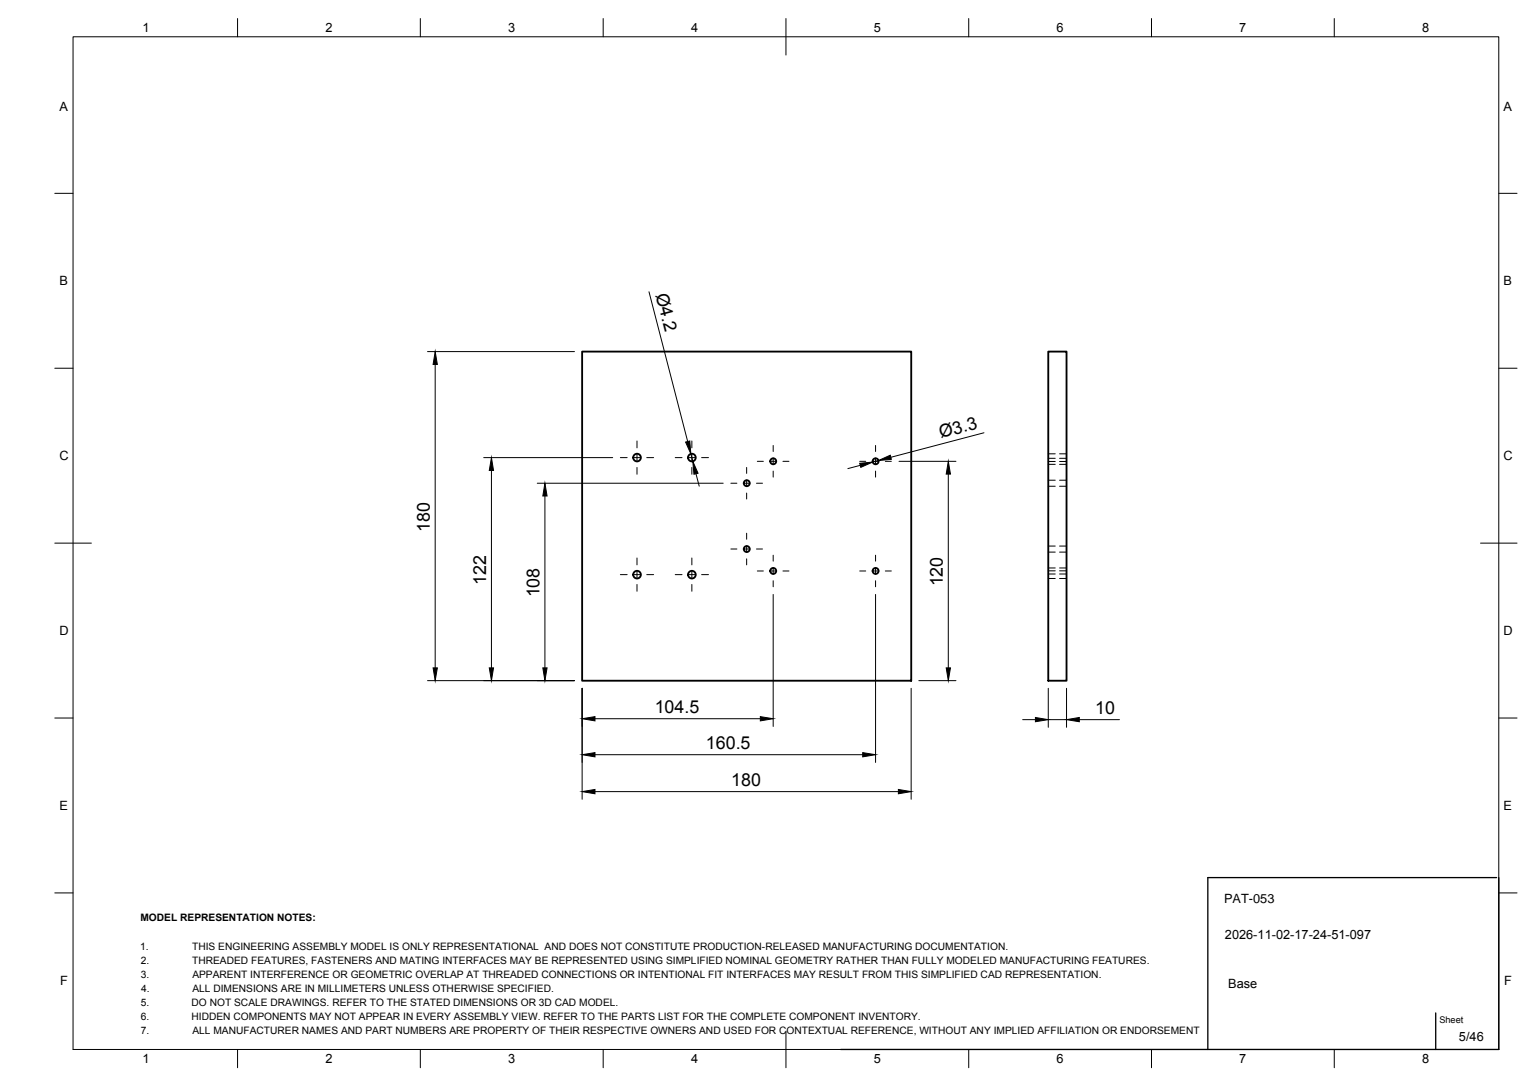
ISO-10303-21;
HEADER;
/* Generated by software containing ST-Developer
 * from STEP Tools, Inc. (www.steptools.com) 
 */

FILE_DESCRIPTION(
/* description */ ('Hand-operated arbor press'),
/* implementation_level */ '2;1');

FILE_NAME(
/* name */ 'Base.step',
/* time_stamp */ '2026-10-28T03:25:25-07:00',
/* author */ (''),
/* organization */ (''),
/* preprocessor_version */ 'ST-DEVELOPER v20.2',
/* originating_system */ 'Autodesk Translation Framework v15.17.0.0',
/* authorisation */ '');

FILE_SCHEMA (('AUTOMOTIVE_DESIGN { 1 0 10303 214 3 1 1 }'));
ENDSEC;

DATA;
#10=MECHANICAL_DESIGN_GEOMETRIC_PRESENTATION_REPRESENTATION('',(#586),#32751);
#502=SHAPE_REPRESENTATION_RELATIONSHIP('SRR','None',#32931,#544);
#544=ADVANCED_BREP_SHAPE_REPRESENTATION('',(#635),#32705);
#586=STYLED_ITEM('',(#33221),#635);
#635=MANIFOLD_SOLID_BREP('Body1',#12483);
#680=FACE_BOUND('',#1989,.T.);
#681=FACE_BOUND('',#1990,.T.);
#682=FACE_BOUND('',#1991,.T.);
#683=FACE_BOUND('',#1992,.T.);
#684=FACE_BOUND('',#1993,.T.);
#685=FACE_BOUND('',#1994,.T.);
#686=FACE_BOUND('',#1995,.T.);
#687=FACE_BOUND('',#1996,.T.);
#688=FACE_BOUND('',#1997,.T.);
#689=FACE_BOUND('',#1998,.T.);
#690=FACE_BOUND('',#2000,.T.);
#691=FACE_BOUND('',#2001,.T.);
#692=FACE_BOUND('',#2002,.T.);
#693=FACE_BOUND('',#2003,.T.);
#694=FACE_BOUND('',#2004,.T.);
#695=FACE_BOUND('',#2005,.T.);
#696=FACE_BOUND('',#2006,.T.);
#697=FACE_BOUND('',#2007,.T.);
#698=FACE_BOUND('',#2008,.T.);
#699=FACE_BOUND('',#2009,.T.);
#849=PLANE('',#13032);
#850=PLANE('',#13033);
#851=PLANE('',#13034);
#852=PLANE('',#13035);
#853=PLANE('',#13036);
#854=PLANE('',#13037);
#1293=FACE_OUTER_BOUND('',#1974,.T.);
#1294=FACE_OUTER_BOUND('',#1975,.T.);
#1295=FACE_OUTER_BOUND('',#1976,.T.);
#1296=FACE_OUTER_BOUND('',#1977,.T.);
#1297=FACE_OUTER_BOUND('',#1978,.T.);
#1298=FACE_OUTER_BOUND('',#1979,.T.);
#1299=FACE_OUTER_BOUND('',#1980,.T.);
#1300=FACE_OUTER_BOUND('',#1981,.T.);
#1301=FACE_OUTER_BOUND('',#1982,.T.);
#1302=FACE_OUTER_BOUND('',#1983,.T.);
#1303=FACE_OUTER_BOUND('',#1984,.T.);
#1304=FACE_OUTER_BOUND('',#1985,.T.);
#1305=FACE_OUTER_BOUND('',#1986,.T.);
#1306=FACE_OUTER_BOUND('',#1987,.T.);
#1307=FACE_OUTER_BOUND('',#1988,.T.);
#1308=FACE_OUTER_BOUND('',#1999,.T.);
#1974=EDGE_LOOP('',(#8324,#8325,#8326,#8327));
#1975=EDGE_LOOP('',(#8328,#8329,#8330,#8331));
#1976=EDGE_LOOP('',(#8332,#8333,#8334,#8335));
#1977=EDGE_LOOP('',(#8336,#8337,#8338,#8339));
#1978=EDGE_LOOP('',(#8340,#8341,#8342,#8343));
#1979=EDGE_LOOP('',(#8344,#8345,#8346,#8347));
#1980=EDGE_LOOP('',(#8348,#8349,#8350,#8351));
#1981=EDGE_LOOP('',(#8352,#8353,#8354,#8355));
#1982=EDGE_LOOP('',(#8356,#8357,#8358,#8359));
#1983=EDGE_LOOP('',(#8360,#8361,#8362,#8363));
#1984=EDGE_LOOP('',(#8364,#8365,#8366,#8367));
#1985=EDGE_LOOP('',(#8368,#8369,#8370,#8371));
#1986=EDGE_LOOP('',(#8372,#8373,#8374,#8375));
#1987=EDGE_LOOP('',(#8376,#8377,#8378,#8379));
#1988=EDGE_LOOP('',(#8380,#8381,#8382,#8383));
#1989=EDGE_LOOP('',(#8384));
#1990=EDGE_LOOP('',(#8385));
#1991=EDGE_LOOP('',(#8386));
#1992=EDGE_LOOP('',(#8387));
#1993=EDGE_LOOP('',(#8388));
#1994=EDGE_LOOP('',(#8389));
#1995=EDGE_LOOP('',(#8390));
#1996=EDGE_LOOP('',(#8391));
#1997=EDGE_LOOP('',(#8392));
#1998=EDGE_LOOP('',(#8393));
#1999=EDGE_LOOP('',(#8394,#8395,#8396,#8397));
#2000=EDGE_LOOP('',(#8398));
#2001=EDGE_LOOP('',(#8399));
#2002=EDGE_LOOP('',(#8400));
#2003=EDGE_LOOP('',(#8401));
#2004=EDGE_LOOP('',(#8402));
#2005=EDGE_LOOP('',(#8403));
#2006=EDGE_LOOP('',(#8404));
#2007=EDGE_LOOP('',(#8405));
#2008=EDGE_LOOP('',(#8406));
#2009=EDGE_LOOP('',(#8407));
#2824=LINE('',#17645,#3995);
#2825=LINE('',#17651,#3996);
#2826=LINE('',#17657,#3997);
#2827=LINE('',#17663,#3998);
#2828=LINE('',#17669,#3999);
#2829=LINE('',#17675,#4000);
#2830=LINE('',#17681,#4001);
#2831=LINE('',#17687,#4002);
#2832=LINE('',#17693,#4003);
#2833=LINE('',#17699,#4004);
#2834=LINE('',#17704,#4005);
#2835=LINE('',#17706,#4006);
#2836=LINE('',#17708,#4007);
#2837=LINE('',#17709,#4008);
#2838=LINE('',#17712,#4009);
#2839=LINE('',#17714,#4010);
#2840=LINE('',#17715,#4011);
#2841=LINE('',#17718,#4012);
#2842=LINE('',#17720,#4013);
#2843=LINE('',#17721,#4014);
#2844=LINE('',#17723,#4015);
#2845=LINE('',#17724,#4016);
#3995=VECTOR('',#14165,0.165);
#3996=VECTOR('',#14172,0.165);
#3997=VECTOR('',#14179,0.165);
#3998=VECTOR('',#14186,0.165);
#3999=VECTOR('',#14193,0.165);
#4000=VECTOR('',#14200,0.165);
#4001=VECTOR('',#14207,0.21);
#4002=VECTOR('',#14214,0.21);
#4003=VECTOR('',#14221,0.21);
#4004=VECTOR('',#14228,0.21);
#4005=VECTOR('',#14233,1.);
#4006=VECTOR('',#14234,1.);
#4007=VECTOR('',#14235,1.);
#4008=VECTOR('',#14236,1.);
#4009=VECTOR('',#14239,1.);
#4010=VECTOR('',#14240,1.);
#4011=VECTOR('',#14241,1.);
#4012=VECTOR('',#14244,1.);
#4013=VECTOR('',#14245,1.);
#4014=VECTOR('',#14246,1.);
#4015=VECTOR('',#14249,1.);
#4016=VECTOR('',#14250,1.);
#5166=CIRCLE('',#13003,0.165);
#5167=CIRCLE('',#13004,0.165);
#5168=CIRCLE('',#13006,0.165);
#5169=CIRCLE('',#13007,0.165);
#5170=CIRCLE('',#13009,0.165);
#5171=CIRCLE('',#13010,0.165);
#5172=CIRCLE('',#13012,0.165);
#5173=CIRCLE('',#13013,0.165);
#5174=CIRCLE('',#13015,0.165);
#5175=CIRCLE('',#13016,0.165);
#5176=CIRCLE('',#13018,0.165);
#5177=CIRCLE('',#13019,0.165);
#5178=CIRCLE('',#13021,0.21);
#5179=CIRCLE('',#13022,0.21);
#5180=CIRCLE('',#13024,0.21);
#5181=CIRCLE('',#13025,0.21);
#5182=CIRCLE('',#13027,0.21);
#5183=CIRCLE('',#13028,0.21);
#5184=CIRCLE('',#13030,0.21);
#5185=CIRCLE('',#13031,0.21);
#5556=VERTEX_POINT('',#17642);
#5557=VERTEX_POINT('',#17644);
#5558=VERTEX_POINT('',#17648);
#5559=VERTEX_POINT('',#17650);
#5560=VERTEX_POINT('',#17654);
#5561=VERTEX_POINT('',#17656);
#5562=VERTEX_POINT('',#17660);
#5563=VERTEX_POINT('',#17662);
#5564=VERTEX_POINT('',#17666);
#5565=VERTEX_POINT('',#17668);
#5566=VERTEX_POINT('',#17672);
#5567=VERTEX_POINT('',#17674);
#5568=VERTEX_POINT('',#17678);
#5569=VERTEX_POINT('',#17680);
#5570=VERTEX_POINT('',#17684);
#5571=VERTEX_POINT('',#17686);
#5572=VERTEX_POINT('',#17690);
#5573=VERTEX_POINT('',#17692);
#5574=VERTEX_POINT('',#17696);
#5575=VERTEX_POINT('',#17698);
#5576=VERTEX_POINT('',#17702);
#5577=VERTEX_POINT('',#17703);
#5578=VERTEX_POINT('',#17705);
#5579=VERTEX_POINT('',#17707);
#5580=VERTEX_POINT('',#17711);
#5581=VERTEX_POINT('',#17713);
#5582=VERTEX_POINT('',#17717);
#5583=VERTEX_POINT('',#17719);
#6665=EDGE_CURVE('',#5556,#5556,#5166,.T.);
#6666=EDGE_CURVE('',#5556,#5557,#2824,.T.);
#6667=EDGE_CURVE('',#5557,#5557,#5167,.T.);
#6668=EDGE_CURVE('',#5558,#5558,#5168,.T.);
#6669=EDGE_CURVE('',#5558,#5559,#2825,.T.);
#6670=EDGE_CURVE('',#5559,#5559,#5169,.T.);
#6671=EDGE_CURVE('',#5560,#5560,#5170,.T.);
#6672=EDGE_CURVE('',#5560,#5561,#2826,.T.);
#6673=EDGE_CURVE('',#5561,#5561,#5171,.T.);
#6674=EDGE_CURVE('',#5562,#5562,#5172,.T.);
#6675=EDGE_CURVE('',#5562,#5563,#2827,.T.);
#6676=EDGE_CURVE('',#5563,#5563,#5173,.T.);
#6677=EDGE_CURVE('',#5564,#5564,#5174,.T.);
#6678=EDGE_CURVE('',#5564,#5565,#2828,.T.);
#6679=EDGE_CURVE('',#5565,#5565,#5175,.T.);
#6680=EDGE_CURVE('',#5566,#5566,#5176,.T.);
#6681=EDGE_CURVE('',#5566,#5567,#2829,.T.);
#6682=EDGE_CURVE('',#5567,#5567,#5177,.T.);
#6683=EDGE_CURVE('',#5568,#5568,#5178,.T.);
#6684=EDGE_CURVE('',#5568,#5569,#2830,.T.);
#6685=EDGE_CURVE('',#5569,#5569,#5179,.T.);
#6686=EDGE_CURVE('',#5570,#5570,#5180,.T.);
#6687=EDGE_CURVE('',#5570,#5571,#2831,.T.);
#6688=EDGE_CURVE('',#5571,#5571,#5181,.T.);
#6689=EDGE_CURVE('',#5572,#5572,#5182,.T.);
#6690=EDGE_CURVE('',#5572,#5573,#2832,.T.);
#6691=EDGE_CURVE('',#5573,#5573,#5183,.T.);
#6692=EDGE_CURVE('',#5574,#5574,#5184,.T.);
#6693=EDGE_CURVE('',#5574,#5575,#2833,.T.);
#6694=EDGE_CURVE('',#5575,#5575,#5185,.T.);
#6695=EDGE_CURVE('',#5576,#5577,#2834,.T.);
#6696=EDGE_CURVE('',#5577,#5578,#2835,.T.);
#6697=EDGE_CURVE('',#5579,#5578,#2836,.T.);
#6698=EDGE_CURVE('',#5576,#5579,#2837,.T.);
#6699=EDGE_CURVE('',#5580,#5576,#2838,.T.);
#6700=EDGE_CURVE('',#5581,#5579,#2839,.T.);
#6701=EDGE_CURVE('',#5580,#5581,#2840,.T.);
#6702=EDGE_CURVE('',#5582,#5580,#2841,.T.);
#6703=EDGE_CURVE('',#5583,#5581,#2842,.T.);
#6704=EDGE_CURVE('',#5582,#5583,#2843,.T.);
#6705=EDGE_CURVE('',#5577,#5582,#2844,.T.);
#6706=EDGE_CURVE('',#5578,#5583,#2845,.T.);
#8324=ORIENTED_EDGE('',*,*,#6665,.F.);
#8325=ORIENTED_EDGE('',*,*,#6666,.T.);
#8326=ORIENTED_EDGE('',*,*,#6667,.F.);
#8327=ORIENTED_EDGE('',*,*,#6666,.F.);
#8328=ORIENTED_EDGE('',*,*,#6668,.F.);
#8329=ORIENTED_EDGE('',*,*,#6669,.T.);
#8330=ORIENTED_EDGE('',*,*,#6670,.F.);
#8331=ORIENTED_EDGE('',*,*,#6669,.F.);
#8332=ORIENTED_EDGE('',*,*,#6671,.F.);
#8333=ORIENTED_EDGE('',*,*,#6672,.T.);
#8334=ORIENTED_EDGE('',*,*,#6673,.F.);
#8335=ORIENTED_EDGE('',*,*,#6672,.F.);
#8336=ORIENTED_EDGE('',*,*,#6674,.F.);
#8337=ORIENTED_EDGE('',*,*,#6675,.T.);
#8338=ORIENTED_EDGE('',*,*,#6676,.F.);
#8339=ORIENTED_EDGE('',*,*,#6675,.F.);
#8340=ORIENTED_EDGE('',*,*,#6677,.F.);
#8341=ORIENTED_EDGE('',*,*,#6678,.T.);
#8342=ORIENTED_EDGE('',*,*,#6679,.F.);
#8343=ORIENTED_EDGE('',*,*,#6678,.F.);
#8344=ORIENTED_EDGE('',*,*,#6680,.F.);
#8345=ORIENTED_EDGE('',*,*,#6681,.T.);
#8346=ORIENTED_EDGE('',*,*,#6682,.F.);
#8347=ORIENTED_EDGE('',*,*,#6681,.F.);
#8348=ORIENTED_EDGE('',*,*,#6683,.F.);
#8349=ORIENTED_EDGE('',*,*,#6684,.T.);
#8350=ORIENTED_EDGE('',*,*,#6685,.F.);
#8351=ORIENTED_EDGE('',*,*,#6684,.F.);
#8352=ORIENTED_EDGE('',*,*,#6686,.F.);
#8353=ORIENTED_EDGE('',*,*,#6687,.T.);
#8354=ORIENTED_EDGE('',*,*,#6688,.F.);
#8355=ORIENTED_EDGE('',*,*,#6687,.F.);
#8356=ORIENTED_EDGE('',*,*,#6689,.F.);
#8357=ORIENTED_EDGE('',*,*,#6690,.T.);
#8358=ORIENTED_EDGE('',*,*,#6691,.F.);
#8359=ORIENTED_EDGE('',*,*,#6690,.F.);
#8360=ORIENTED_EDGE('',*,*,#6692,.F.);
#8361=ORIENTED_EDGE('',*,*,#6693,.T.);
#8362=ORIENTED_EDGE('',*,*,#6694,.F.);
#8363=ORIENTED_EDGE('',*,*,#6693,.F.);
#8364=ORIENTED_EDGE('',*,*,#6695,.T.);
#8365=ORIENTED_EDGE('',*,*,#6696,.T.);
#8366=ORIENTED_EDGE('',*,*,#6697,.F.);
#8367=ORIENTED_EDGE('',*,*,#6698,.F.);
#8368=ORIENTED_EDGE('',*,*,#6699,.T.);
#8369=ORIENTED_EDGE('',*,*,#6698,.T.);
#8370=ORIENTED_EDGE('',*,*,#6700,.F.);
#8371=ORIENTED_EDGE('',*,*,#6701,.F.);
#8372=ORIENTED_EDGE('',*,*,#6702,.T.);
#8373=ORIENTED_EDGE('',*,*,#6701,.T.);
#8374=ORIENTED_EDGE('',*,*,#6703,.F.);
#8375=ORIENTED_EDGE('',*,*,#6704,.F.);
#8376=ORIENTED_EDGE('',*,*,#6705,.T.);
#8377=ORIENTED_EDGE('',*,*,#6704,.T.);
#8378=ORIENTED_EDGE('',*,*,#6706,.F.);
#8379=ORIENTED_EDGE('',*,*,#6696,.F.);
#8380=ORIENTED_EDGE('',*,*,#6706,.T.);
#8381=ORIENTED_EDGE('',*,*,#6703,.T.);
#8382=ORIENTED_EDGE('',*,*,#6700,.T.);
#8383=ORIENTED_EDGE('',*,*,#6697,.T.);
#8384=ORIENTED_EDGE('',*,*,#6673,.T.);
#8385=ORIENTED_EDGE('',*,*,#6676,.T.);
#8386=ORIENTED_EDGE('',*,*,#6679,.T.);
#8387=ORIENTED_EDGE('',*,*,#6682,.T.);
#8388=ORIENTED_EDGE('',*,*,#6685,.T.);
#8389=ORIENTED_EDGE('',*,*,#6688,.T.);
#8390=ORIENTED_EDGE('',*,*,#6691,.T.);
#8391=ORIENTED_EDGE('',*,*,#6694,.T.);
#8392=ORIENTED_EDGE('',*,*,#6670,.T.);
#8393=ORIENTED_EDGE('',*,*,#6667,.T.);
#8394=ORIENTED_EDGE('',*,*,#6705,.F.);
#8395=ORIENTED_EDGE('',*,*,#6695,.F.);
#8396=ORIENTED_EDGE('',*,*,#6699,.F.);
#8397=ORIENTED_EDGE('',*,*,#6702,.F.);
#8398=ORIENTED_EDGE('',*,*,#6671,.T.);
#8399=ORIENTED_EDGE('',*,*,#6674,.T.);
#8400=ORIENTED_EDGE('',*,*,#6677,.T.);
#8401=ORIENTED_EDGE('',*,*,#6680,.T.);
#8402=ORIENTED_EDGE('',*,*,#6683,.T.);
#8403=ORIENTED_EDGE('',*,*,#6686,.T.);
#8404=ORIENTED_EDGE('',*,*,#6689,.T.);
#8405=ORIENTED_EDGE('',*,*,#6692,.T.);
#8406=ORIENTED_EDGE('',*,*,#6668,.T.);
#8407=ORIENTED_EDGE('',*,*,#6665,.T.);
#11642=CYLINDRICAL_SURFACE('',#13002,0.165);
#11643=CYLINDRICAL_SURFACE('',#13005,0.165);
#11644=CYLINDRICAL_SURFACE('',#13008,0.165);
#11645=CYLINDRICAL_SURFACE('',#13011,0.165);
#11646=CYLINDRICAL_SURFACE('',#13014,0.165);
#11647=CYLINDRICAL_SURFACE('',#13017,0.165);
#11648=CYLINDRICAL_SURFACE('',#13020,0.21);
#11649=CYLINDRICAL_SURFACE('',#13023,0.21);
#11650=CYLINDRICAL_SURFACE('',#13026,0.21);
#11651=CYLINDRICAL_SURFACE('',#13029,0.21);
#11802=ADVANCED_FACE('',(#1293),#11642,.F.);
#11803=ADVANCED_FACE('',(#1294),#11643,.F.);
#11804=ADVANCED_FACE('',(#1295),#11644,.F.);
#11805=ADVANCED_FACE('',(#1296),#11645,.F.);
#11806=ADVANCED_FACE('',(#1297),#11646,.F.);
#11807=ADVANCED_FACE('',(#1298),#11647,.F.);
#11808=ADVANCED_FACE('',(#1299),#11648,.F.);
#11809=ADVANCED_FACE('',(#1300),#11649,.F.);
#11810=ADVANCED_FACE('',(#1301),#11650,.F.);
#11811=ADVANCED_FACE('',(#1302),#11651,.F.);
#11812=ADVANCED_FACE('',(#1303),#849,.T.);
#11813=ADVANCED_FACE('',(#1304),#850,.T.);
#11814=ADVANCED_FACE('',(#1305),#851,.T.);
#11815=ADVANCED_FACE('',(#1306),#852,.T.);
#11816=ADVANCED_FACE('',(#1307,#680,#681,#682,#683,#684,#685,#686,#687,
#688,#689),#853,.T.);
#11817=ADVANCED_FACE('',(#1308,#690,#691,#692,#693,#694,#695,#696,#697,
#698,#699),#854,.F.);
#12483=CLOSED_SHELL('',(#11802,#11803,#11804,#11805,#11806,#11807,#11808,
#11809,#11810,#11811,#11812,#11813,#11814,#11815,#11816,#11817));
#13001=AXIS2_PLACEMENT_3D('',#17640,#14159,#14160);
#13002=AXIS2_PLACEMENT_3D('',#17641,#14161,#14162);
#13003=AXIS2_PLACEMENT_3D('',#17643,#14163,#14164);
#13004=AXIS2_PLACEMENT_3D('',#17646,#14166,#14167);
#13005=AXIS2_PLACEMENT_3D('',#17647,#14168,#14169);
#13006=AXIS2_PLACEMENT_3D('',#17649,#14170,#14171);
#13007=AXIS2_PLACEMENT_3D('',#17652,#14173,#14174);
#13008=AXIS2_PLACEMENT_3D('',#17653,#14175,#14176);
#13009=AXIS2_PLACEMENT_3D('',#17655,#14177,#14178);
#13010=AXIS2_PLACEMENT_3D('',#17658,#14180,#14181);
#13011=AXIS2_PLACEMENT_3D('',#17659,#14182,#14183);
#13012=AXIS2_PLACEMENT_3D('',#17661,#14184,#14185);
#13013=AXIS2_PLACEMENT_3D('',#17664,#14187,#14188);
#13014=AXIS2_PLACEMENT_3D('',#17665,#14189,#14190);
#13015=AXIS2_PLACEMENT_3D('',#17667,#14191,#14192);
#13016=AXIS2_PLACEMENT_3D('',#17670,#14194,#14195);
#13017=AXIS2_PLACEMENT_3D('',#17671,#14196,#14197);
#13018=AXIS2_PLACEMENT_3D('',#17673,#14198,#14199);
#13019=AXIS2_PLACEMENT_3D('',#17676,#14201,#14202);
#13020=AXIS2_PLACEMENT_3D('',#17677,#14203,#14204);
#13021=AXIS2_PLACEMENT_3D('',#17679,#14205,#14206);
#13022=AXIS2_PLACEMENT_3D('',#17682,#14208,#14209);
#13023=AXIS2_PLACEMENT_3D('',#17683,#14210,#14211);
#13024=AXIS2_PLACEMENT_3D('',#17685,#14212,#14213);
#13025=AXIS2_PLACEMENT_3D('',#17688,#14215,#14216);
#13026=AXIS2_PLACEMENT_3D('',#17689,#14217,#14218);
#13027=AXIS2_PLACEMENT_3D('',#17691,#14219,#14220);
#13028=AXIS2_PLACEMENT_3D('',#17694,#14222,#14223);
#13029=AXIS2_PLACEMENT_3D('',#17695,#14224,#14225);
#13030=AXIS2_PLACEMENT_3D('',#17697,#14226,#14227);
#13031=AXIS2_PLACEMENT_3D('',#17700,#14229,#14230);
#13032=AXIS2_PLACEMENT_3D('',#17701,#14231,#14232);
#13033=AXIS2_PLACEMENT_3D('',#17710,#14237,#14238);
#13034=AXIS2_PLACEMENT_3D('',#17716,#14242,#14243);
#13035=AXIS2_PLACEMENT_3D('',#17722,#14247,#14248);
#13036=AXIS2_PLACEMENT_3D('',#17725,#14251,#14252);
#13037=AXIS2_PLACEMENT_3D('',#17726,#14253,#14254);
#14159=DIRECTION('axis',(0.,0.,1.));
#14160=DIRECTION('refdir',(1.,0.,0.));
#14161=DIRECTION('center_axis',(0.,0.,1.));
#14162=DIRECTION('ref_axis',(1.,0.,0.));
#14163=DIRECTION('center_axis',(0.,0.,1.));
#14164=DIRECTION('ref_axis',(1.,0.,0.));
#14165=DIRECTION('',(0.,0.,1.));
#14166=DIRECTION('center_axis',(0.,0.,-1.));
#14167=DIRECTION('ref_axis',(1.,0.,0.));
#14168=DIRECTION('center_axis',(0.,0.,1.));
#14169=DIRECTION('ref_axis',(1.,0.,0.));
#14170=DIRECTION('center_axis',(0.,0.,1.));
#14171=DIRECTION('ref_axis',(1.,0.,0.));
#14172=DIRECTION('',(0.,0.,1.));
#14173=DIRECTION('center_axis',(0.,0.,-1.));
#14174=DIRECTION('ref_axis',(1.,0.,0.));
#14175=DIRECTION('center_axis',(0.,0.,1.));
#14176=DIRECTION('ref_axis',(1.,0.,0.));
#14177=DIRECTION('center_axis',(0.,0.,1.));
#14178=DIRECTION('ref_axis',(1.,0.,0.));
#14179=DIRECTION('',(0.,0.,1.));
#14180=DIRECTION('center_axis',(0.,0.,-1.));
#14181=DIRECTION('ref_axis',(1.,0.,0.));
#14182=DIRECTION('center_axis',(0.,0.,1.));
#14183=DIRECTION('ref_axis',(1.,0.,0.));
#14184=DIRECTION('center_axis',(0.,0.,1.));
#14185=DIRECTION('ref_axis',(1.,0.,0.));
#14186=DIRECTION('',(0.,0.,1.));
#14187=DIRECTION('center_axis',(0.,0.,-1.));
#14188=DIRECTION('ref_axis',(1.,0.,0.));
#14189=DIRECTION('center_axis',(0.,0.,1.));
#14190=DIRECTION('ref_axis',(1.,0.,0.));
#14191=DIRECTION('center_axis',(0.,0.,1.));
#14192=DIRECTION('ref_axis',(1.,0.,0.));
#14193=DIRECTION('',(0.,0.,1.));
#14194=DIRECTION('center_axis',(0.,0.,-1.));
#14195=DIRECTION('ref_axis',(1.,0.,0.));
#14196=DIRECTION('center_axis',(0.,0.,1.));
#14197=DIRECTION('ref_axis',(1.,0.,0.));
#14198=DIRECTION('center_axis',(0.,0.,1.));
#14199=DIRECTION('ref_axis',(1.,0.,0.));
#14200=DIRECTION('',(0.,0.,1.));
#14201=DIRECTION('center_axis',(0.,0.,-1.));
#14202=DIRECTION('ref_axis',(1.,0.,0.));
#14203=DIRECTION('center_axis',(0.,0.,1.));
#14204=DIRECTION('ref_axis',(1.,0.,0.));
#14205=DIRECTION('center_axis',(0.,0.,1.));
#14206=DIRECTION('ref_axis',(1.,0.,0.));
#14207=DIRECTION('',(0.,0.,1.));
#14208=DIRECTION('center_axis',(0.,0.,-1.));
#14209=DIRECTION('ref_axis',(1.,0.,0.));
#14210=DIRECTION('center_axis',(0.,0.,1.));
#14211=DIRECTION('ref_axis',(1.,0.,0.));
#14212=DIRECTION('center_axis',(0.,0.,1.));
#14213=DIRECTION('ref_axis',(1.,0.,0.));
#14214=DIRECTION('',(0.,0.,1.));
#14215=DIRECTION('center_axis',(0.,0.,-1.));
#14216=DIRECTION('ref_axis',(1.,0.,0.));
#14217=DIRECTION('center_axis',(0.,0.,1.));
#14218=DIRECTION('ref_axis',(1.,0.,0.));
#14219=DIRECTION('center_axis',(0.,0.,1.));
#14220=DIRECTION('ref_axis',(1.,0.,0.));
#14221=DIRECTION('',(0.,0.,1.));
#14222=DIRECTION('center_axis',(0.,0.,-1.));
#14223=DIRECTION('ref_axis',(1.,0.,0.));
#14224=DIRECTION('center_axis',(0.,0.,1.));
#14225=DIRECTION('ref_axis',(1.,0.,0.));
#14226=DIRECTION('center_axis',(0.,0.,1.));
#14227=DIRECTION('ref_axis',(1.,0.,0.));
#14228=DIRECTION('',(0.,0.,1.));
#14229=DIRECTION('center_axis',(0.,0.,-1.));
#14230=DIRECTION('ref_axis',(1.,0.,0.));
#14231=DIRECTION('center_axis',(0.,1.,0.));
#14232=DIRECTION('ref_axis',(-1.,0.,0.));
#14233=DIRECTION('',(-1.,0.,0.));
#14234=DIRECTION('',(0.,0.,1.));
#14235=DIRECTION('',(-1.,0.,0.));
#14236=DIRECTION('',(0.,0.,1.));
#14237=DIRECTION('center_axis',(1.,0.,0.));
#14238=DIRECTION('ref_axis',(0.,1.,0.));
#14239=DIRECTION('',(0.,1.,0.));
#14240=DIRECTION('',(0.,1.,0.));
#14241=DIRECTION('',(0.,0.,1.));
#14242=DIRECTION('center_axis',(0.,-1.,0.));
#14243=DIRECTION('ref_axis',(1.,0.,0.));
#14244=DIRECTION('',(1.,0.,0.));
#14245=DIRECTION('',(1.,0.,0.));
#14246=DIRECTION('',(0.,0.,1.));
#14247=DIRECTION('center_axis',(-1.,0.,0.));
#14248=DIRECTION('ref_axis',(0.,-1.,0.));
#14249=DIRECTION('',(0.,-1.,0.));
#14250=DIRECTION('',(0.,-1.,0.));
#14251=DIRECTION('center_axis',(0.,0.,1.));
#14252=DIRECTION('ref_axis',(1.,0.,0.));
#14253=DIRECTION('center_axis',(0.,0.,1.));
#14254=DIRECTION('ref_axis',(1.,0.,0.));
#17640=CARTESIAN_POINT('',(0.,0.,0.));
#17641=CARTESIAN_POINT('Origin',(-6.05,3.,-0.1));
#17642=CARTESIAN_POINT('',(-6.215,3.,0.));
#17643=CARTESIAN_POINT('Origin',(-6.05,3.,0.));
#17644=CARTESIAN_POINT('',(-6.215,3.,1.));
#17645=CARTESIAN_POINT('',(-6.215,3.,-0.1));
#17646=CARTESIAN_POINT('Origin',(-6.05,3.,1.));
#17647=CARTESIAN_POINT('Origin',(-0.45,3.,-0.1));
#17648=CARTESIAN_POINT('',(-0.615,3.,0.));
#17649=CARTESIAN_POINT('Origin',(-0.45,3.,0.));
#17650=CARTESIAN_POINT('',(-0.615,3.,1.));
#17651=CARTESIAN_POINT('',(-0.615,3.,-0.1));
#17652=CARTESIAN_POINT('Origin',(-0.45,3.,1.));
#17653=CARTESIAN_POINT('Origin',(-6.05,-3.,-0.1));
#17654=CARTESIAN_POINT('',(-6.215,-3.,0.));
#17655=CARTESIAN_POINT('Origin',(-6.05,-3.,0.));
#17656=CARTESIAN_POINT('',(-6.215,-3.,1.));
#17657=CARTESIAN_POINT('',(-6.215,-3.,-0.1));
#17658=CARTESIAN_POINT('Origin',(-6.05,-3.,1.));
#17659=CARTESIAN_POINT('Origin',(-0.45,-3.,-0.1));
#17660=CARTESIAN_POINT('',(-0.615,-3.,0.));
#17661=CARTESIAN_POINT('Origin',(-0.45,-3.,0.));
#17662=CARTESIAN_POINT('',(-0.615,-3.,1.));
#17663=CARTESIAN_POINT('',(-0.615,-3.,-0.1));
#17664=CARTESIAN_POINT('Origin',(-0.45,-3.,1.));
#17665=CARTESIAN_POINT('Origin',(1.,-1.8,-0.1));
#17666=CARTESIAN_POINT('',(0.835,-1.8,0.));
#17667=CARTESIAN_POINT('Origin',(1.,-1.8,0.));
#17668=CARTESIAN_POINT('',(0.835,-1.8,1.));
#17669=CARTESIAN_POINT('',(0.835,-1.8,-0.1));
#17670=CARTESIAN_POINT('Origin',(1.,-1.8,1.));
#17671=CARTESIAN_POINT('Origin',(1.,1.8,-0.1));
#17672=CARTESIAN_POINT('',(0.835,1.8,0.));
#17673=CARTESIAN_POINT('Origin',(1.,1.8,0.));
#17674=CARTESIAN_POINT('',(0.835,1.8,1.));
#17675=CARTESIAN_POINT('',(0.835,1.8,-0.1));
#17676=CARTESIAN_POINT('Origin',(1.,1.8,1.));
#17677=CARTESIAN_POINT('Origin',(7.,-3.2,-0.1));
#17678=CARTESIAN_POINT('',(6.79,-3.2,0.));
#17679=CARTESIAN_POINT('Origin',(7.,-3.2,0.));
#17680=CARTESIAN_POINT('',(6.79,-3.2,1.));
#17681=CARTESIAN_POINT('',(6.79,-3.2,-0.1));
#17682=CARTESIAN_POINT('Origin',(7.,-3.2,1.));
#17683=CARTESIAN_POINT('Origin',(4.,3.2,-0.1));
#17684=CARTESIAN_POINT('',(3.79,3.2,0.));
#17685=CARTESIAN_POINT('Origin',(4.,3.2,0.));
#17686=CARTESIAN_POINT('',(3.79,3.2,1.));
#17687=CARTESIAN_POINT('',(3.79,3.2,-0.1));
#17688=CARTESIAN_POINT('Origin',(4.,3.2,1.));
#17689=CARTESIAN_POINT('Origin',(4.,-3.2,-0.1));
#17690=CARTESIAN_POINT('',(3.79,-3.2,0.));
#17691=CARTESIAN_POINT('Origin',(4.,-3.2,0.));
#17692=CARTESIAN_POINT('',(3.79,-3.2,1.));
#17693=CARTESIAN_POINT('',(3.79,-3.2,-0.1));
#17694=CARTESIAN_POINT('Origin',(4.,-3.2,1.));
#17695=CARTESIAN_POINT('Origin',(7.,3.2,-0.1));
#17696=CARTESIAN_POINT('',(6.79,3.2,0.));
#17697=CARTESIAN_POINT('Origin',(7.,3.2,0.));
#17698=CARTESIAN_POINT('',(6.79,3.2,1.));
#17699=CARTESIAN_POINT('',(6.79,3.2,-0.1));
#17700=CARTESIAN_POINT('Origin',(7.,3.2,1.));
#17701=CARTESIAN_POINT('Origin',(10.,9.,0.));
#17702=CARTESIAN_POINT('',(10.,9.,0.));
#17703=CARTESIAN_POINT('',(-8.,9.,0.));
#17704=CARTESIAN_POINT('',(10.,9.,0.));
#17705=CARTESIAN_POINT('',(-8.,9.,1.));
#17706=CARTESIAN_POINT('',(-8.,9.,0.));
#17707=CARTESIAN_POINT('',(10.,9.,1.));
#17708=CARTESIAN_POINT('',(10.,9.,1.));
#17709=CARTESIAN_POINT('',(10.,9.,0.));
#17710=CARTESIAN_POINT('Origin',(10.,-9.,0.));
#17711=CARTESIAN_POINT('',(10.,-9.,0.));
#17712=CARTESIAN_POINT('',(10.,-9.,0.));
#17713=CARTESIAN_POINT('',(10.,-9.,1.));
#17714=CARTESIAN_POINT('',(10.,-9.,1.));
#17715=CARTESIAN_POINT('',(10.,-9.,0.));
#17716=CARTESIAN_POINT('Origin',(-8.,-9.,0.));
#17717=CARTESIAN_POINT('',(-8.,-9.,0.));
#17718=CARTESIAN_POINT('',(-8.,-9.,0.));
#17719=CARTESIAN_POINT('',(-8.,-9.,1.));
#17720=CARTESIAN_POINT('',(-8.,-9.,1.));
#17721=CARTESIAN_POINT('',(-8.,-9.,0.));
#17722=CARTESIAN_POINT('Origin',(-8.,9.,0.));
#17723=CARTESIAN_POINT('',(-8.,9.,0.));
#17724=CARTESIAN_POINT('',(-8.,9.,1.));
#17725=CARTESIAN_POINT('Origin',(1.,0.,1.));
#17726=CARTESIAN_POINT('Origin',(1.,0.,0.));
#32656=UNCERTAINTY_MEASURE_WITH_UNIT(LENGTH_MEASURE(0.001),#32752,
'DISTANCE_ACCURACY_VALUE',
'Maximum model space distance between geometric entities at asserted c
onnectivities');
#32702=UNCERTAINTY_MEASURE_WITH_UNIT(LENGTH_MEASURE(0.001),#32752,
'DISTANCE_ACCURACY_VALUE',
'Maximum model space distance between geometric entities at asserted c
onnectivities');
#32705=(
GEOMETRIC_REPRESENTATION_CONTEXT(3)
GLOBAL_UNCERTAINTY_ASSIGNED_CONTEXT((#32656))
GLOBAL_UNIT_ASSIGNED_CONTEXT((#32752,#32754,#32755))
REPRESENTATION_CONTEXT('','3D')
);
#32751=(
GEOMETRIC_REPRESENTATION_CONTEXT(3)
GLOBAL_UNCERTAINTY_ASSIGNED_CONTEXT((#32702))
GLOBAL_UNIT_ASSIGNED_CONTEXT((#32752,#32754,#32755))
REPRESENTATION_CONTEXT('','3D')
);
#32752=(
LENGTH_UNIT()
NAMED_UNIT(*)
SI_UNIT(.CENTI.,.METRE.)
);
#32754=(
NAMED_UNIT(*)
PLANE_ANGLE_UNIT()
SI_UNIT($,.RADIAN.)
);
#32755=(
NAMED_UNIT(*)
SI_UNIT($,.STERADIAN.)
SOLID_ANGLE_UNIT()
);
#32758=SHAPE_DEFINITION_REPRESENTATION(#32806,#32931);
#32806=PRODUCT_DEFINITION_SHAPE('',$,#32980);
#32931=SHAPE_REPRESENTATION('',(#13001),#32705);
#32977=PRODUCT_DEFINITION_CONTEXT('part definition',#33123,'design');
#32980=PRODUCT_DEFINITION('Base','Base',#33028,#32977);
#33028=PRODUCT_DEFINITION_FORMATION('',$,#33127);
#33123=APPLICATION_CONTEXT(
'Core Data for Automotive Mechanical Design Process');
#33124=PRODUCT_CONTEXT('part definition',#33123,'mechanical');
#33127=PRODUCT('Base','Base','Base',(#33124));
#33215=COLOUR_RGB('Dark Blue',0.08,0.2,0.34);
#33216=FILL_AREA_STYLE_COLOUR('',#33215);
#33217=FILL_AREA_STYLE('',(#33216));
#33218=SURFACE_STYLE_FILL_AREA(#33217);
#33219=SURFACE_SIDE_STYLE('',(#33218));
#33220=SURFACE_STYLE_USAGE(.BOTH.,#33219);
#33221=PRESENTATION_STYLE_ASSIGNMENT((#33220));
ENDSEC;
END-ISO-10303-21;
